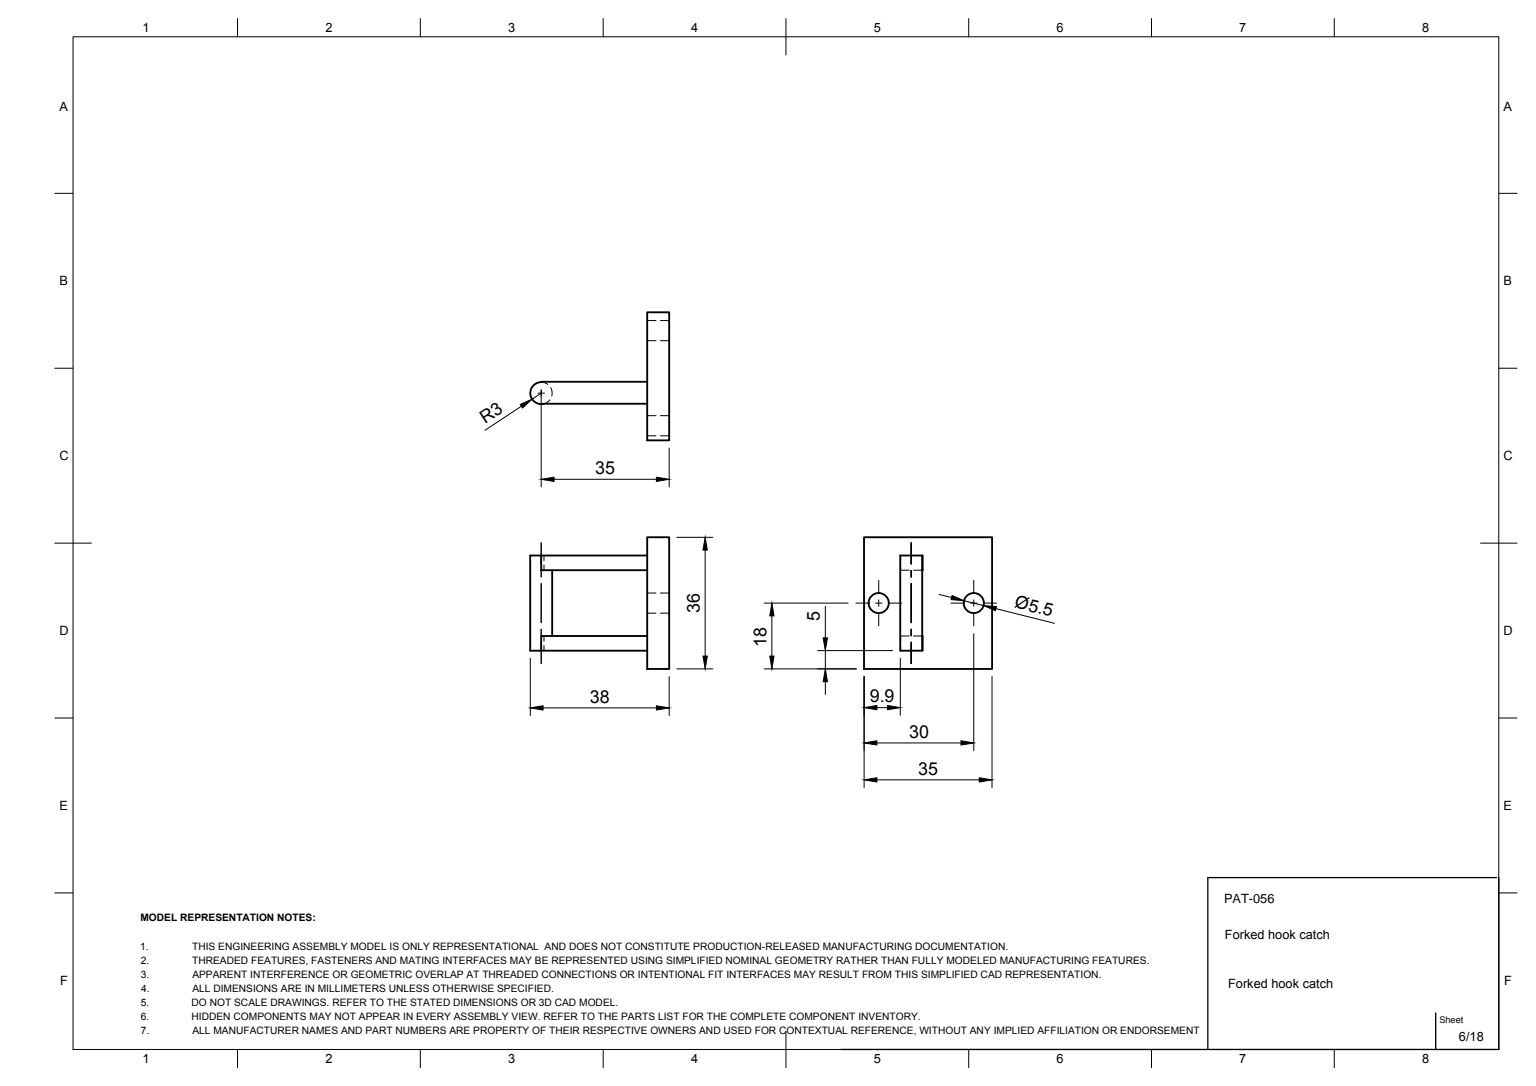
ISO-10303-21;
HEADER;
/* Generated by software containing ST-Developer
 * from STEP Tools, Inc. (www.steptools.com) 
 */

FILE_DESCRIPTION(
/* description */ ('Hook toggle clamp'),
/* implementation_level */ '2;1');

FILE_NAME(
/* name */ 'Forked hook catch.step',
/* time_stamp */ '2026-10-27T21:56:56-07:00',
/* author */ (''),
/* organization */ (''),
/* preprocessor_version */ 'ST-DEVELOPER v20.2',
/* originating_system */ 'Autodesk Translation Framework v15.17.0.0',
/* authorisation */ '');

FILE_SCHEMA (('AUTOMOTIVE_DESIGN { 1 0 10303 214 3 1 1 }'));
ENDSEC;

DATA;
#10=MECHANICAL_DESIGN_GEOMETRIC_PRESENTATION_REPRESENTATION('',(#191),#5458);
#157=SHAPE_REPRESENTATION_RELATIONSHIP('SRR','None',#5538,#174);
#174=ADVANCED_BREP_SHAPE_REPRESENTATION('',(#208),#5440);
#191=STYLED_ITEM('',(#5731),#208);
#208=MANIFOLD_SOLID_BREP('Body1',#2972);
#237=FACE_BOUND('',#641,.T.);
#238=FACE_BOUND('',#642,.T.);
#239=FACE_BOUND('',#643,.T.);
#240=FACE_BOUND('',#644,.T.);
#241=FACE_BOUND('',#646,.T.);
#242=FACE_BOUND('',#647,.T.);
#312=PLANE('',#3244);
#313=PLANE('',#3252);
#314=PLANE('',#3253);
#315=PLANE('',#3254);
#316=PLANE('',#3255);
#317=PLANE('',#3256);
#318=PLANE('',#3257);
#319=PLANE('',#3258);
#320=PLANE('',#3259);
#321=PLANE('',#3260);
#322=PLANE('',#3261);
#323=PLANE('',#3262);
#324=PLANE('',#3263);
#325=PLANE('',#3264);
#326=PLANE('',#3265);
#327=PLANE('',#3266);
#435=FACE_OUTER_BOUND('',#623,.T.);
#436=FACE_OUTER_BOUND('',#624,.T.);
#437=FACE_OUTER_BOUND('',#625,.T.);
#438=FACE_OUTER_BOUND('',#626,.T.);
#439=FACE_OUTER_BOUND('',#627,.T.);
#440=FACE_OUTER_BOUND('',#628,.T.);
#441=FACE_OUTER_BOUND('',#629,.T.);
#442=FACE_OUTER_BOUND('',#630,.T.);
#443=FACE_OUTER_BOUND('',#631,.T.);
#444=FACE_OUTER_BOUND('',#632,.T.);
#445=FACE_OUTER_BOUND('',#633,.T.);
#446=FACE_OUTER_BOUND('',#634,.T.);
#447=FACE_OUTER_BOUND('',#635,.T.);
#448=FACE_OUTER_BOUND('',#636,.T.);
#449=FACE_OUTER_BOUND('',#637,.T.);
#450=FACE_OUTER_BOUND('',#638,.T.);
#451=FACE_OUTER_BOUND('',#639,.T.);
#452=FACE_OUTER_BOUND('',#640,.T.);
#453=FACE_OUTER_BOUND('',#645,.T.);
#623=EDGE_LOOP('',(#2197,#2198,#2199,#2200));
#624=EDGE_LOOP('',(#2201,#2202,#2203,#2204));
#625=EDGE_LOOP('',(#2205,#2206,#2207,#2208,#2209));
#626=EDGE_LOOP('',(#2210,#2211,#2212,#2213,#2214,#2215,#2216,#2217,#2218,
#2219,#2220,#2221));
#627=EDGE_LOOP('',(#2222,#2223,#2224,#2225,#2226,#2227));
#628=EDGE_LOOP('',(#2228,#2229,#2230,#2231));
#629=EDGE_LOOP('',(#2232,#2233,#2234,#2235));
#630=EDGE_LOOP('',(#2236,#2237,#2238,#2239));
#631=EDGE_LOOP('',(#2240,#2241,#2242,#2243,#2244));
#632=EDGE_LOOP('',(#2245,#2246,#2247,#2248));
#633=EDGE_LOOP('',(#2249,#2250,#2251,#2252,#2253,#2254));
#634=EDGE_LOOP('',(#2255,#2256,#2257,#2258));
#635=EDGE_LOOP('',(#2259,#2260,#2261,#2262));
#636=EDGE_LOOP('',(#2263,#2264,#2265,#2266));
#637=EDGE_LOOP('',(#2267,#2268,#2269,#2270));
#638=EDGE_LOOP('',(#2271,#2272,#2273,#2274));
#639=EDGE_LOOP('',(#2275,#2276,#2277,#2278));
#640=EDGE_LOOP('',(#2279,#2280,#2281,#2282));
#641=EDGE_LOOP('',(#2283));
#642=EDGE_LOOP('',(#2284));
#643=EDGE_LOOP('',(#2285,#2286,#2287,#2288));
#644=EDGE_LOOP('',(#2289,#2290,#2291,#2292));
#645=EDGE_LOOP('',(#2293,#2294,#2295,#2296));
#646=EDGE_LOOP('',(#2297));
#647=EDGE_LOOP('',(#2298));
#872=LINE('',#4644,#1109);
#873=LINE('',#4650,#1110);
#874=LINE('',#4657,#1111);
#875=LINE('',#4659,#1112);
#876=LINE('',#4661,#1113);
#877=LINE('',#4662,#1114);
#878=LINE('',#4665,#1115);
#879=LINE('',#4667,#1116);
#880=LINE('',#4671,#1117);
#881=LINE('',#4675,#1118);
#882=LINE('',#4679,#1119);
#883=LINE('',#4684,#1120);
#884=LINE('',#4686,#1121);
#885=LINE('',#4688,#1122);
#886=LINE('',#4689,#1123);
#887=LINE('',#4691,#1124);
#888=LINE('',#4693,#1125);
#889=LINE('',#4695,#1126);
#890=LINE('',#4698,#1127);
#891=LINE('',#4700,#1128);
#892=LINE('',#4702,#1129);
#893=LINE('',#4703,#1130);
#894=LINE('',#4706,#1131);
#895=LINE('',#4707,#1132);
#896=LINE('',#4710,#1133);
#897=LINE('',#4712,#1134);
#898=LINE('',#4713,#1135);
#899=LINE('',#4715,#1136);
#900=LINE('',#4717,#1137);
#901=LINE('',#4721,#1138);
#902=LINE('',#4723,#1139);
#903=LINE('',#4725,#1140);
#904=LINE('',#4726,#1141);
#905=LINE('',#4729,#1142);
#906=LINE('',#4731,#1143);
#907=LINE('',#4732,#1144);
#908=LINE('',#4735,#1145);
#909=LINE('',#4737,#1146);
#910=LINE('',#4738,#1147);
#911=LINE('',#4740,#1148);
#912=LINE('',#4741,#1149);
#1109=VECTOR('',#3716,0.275);
#1110=VECTOR('',#3723,0.274999999999999);
#1111=VECTOR('',#3730,1.);
#1112=VECTOR('',#3731,1.);
#1113=VECTOR('',#3732,1.);
#1114=VECTOR('',#3733,1.);
#1115=VECTOR('',#3736,1.);
#1116=VECTOR('',#3737,1.);
#1117=VECTOR('',#3740,0.300000000000001);
#1118=VECTOR('',#3743,1.);
#1119=VECTOR('',#3746,1.);
#1120=VECTOR('',#3753,1.);
#1121=VECTOR('',#3754,1.);
#1122=VECTOR('',#3755,1.);
#1123=VECTOR('',#3756,1.);
#1124=VECTOR('',#3759,1.);
#1125=VECTOR('',#3762,1.);
#1126=VECTOR('',#3765,1.);
#1127=VECTOR('',#3768,1.);
#1128=VECTOR('',#3769,1.);
#1129=VECTOR('',#3770,1.);
#1130=VECTOR('',#3771,1.);
#1131=VECTOR('',#3774,1.);
#1132=VECTOR('',#3775,1.);
#1133=VECTOR('',#3778,1.);
#1134=VECTOR('',#3779,1.);
#1135=VECTOR('',#3780,1.);
#1136=VECTOR('',#3783,1.);
#1137=VECTOR('',#3786,1.);
#1138=VECTOR('',#3789,1.);
#1139=VECTOR('',#3790,1.);
#1140=VECTOR('',#3791,1.);
#1141=VECTOR('',#3792,1.);
#1142=VECTOR('',#3795,1.);
#1143=VECTOR('',#3796,1.);
#1144=VECTOR('',#3797,1.);
#1145=VECTOR('',#3800,1.);
#1146=VECTOR('',#3801,1.);
#1147=VECTOR('',#3802,1.);
#1148=VECTOR('',#3805,1.);
#1149=VECTOR('',#3806,1.);
#1284=CIRCLE('',#3239,0.275);
#1285=CIRCLE('',#3240,0.275);
#1286=CIRCLE('',#3242,0.274999999999999);
#1287=CIRCLE('',#3243,0.274999999999999);
#1288=CIRCLE('',#3245,0.300000000000001);
#1289=CIRCLE('',#3247,0.300000000000001);
#1290=CIRCLE('',#3248,0.300000000000001);
#1291=CIRCLE('',#3249,0.300000000000001);
#1292=CIRCLE('',#3250,0.300000000000001);
#1293=CIRCLE('',#3251,0.300000000000001);
#1447=VERTEX_POINT('',#4641);
#1448=VERTEX_POINT('',#4643);
#1449=VERTEX_POINT('',#4647);
#1450=VERTEX_POINT('',#4649);
#1451=VERTEX_POINT('',#4653);
#1452=VERTEX_POINT('',#4654);
#1453=VERTEX_POINT('',#4656);
#1454=VERTEX_POINT('',#4658);
#1455=VERTEX_POINT('',#4660);
#1456=VERTEX_POINT('',#4664);
#1457=VERTEX_POINT('',#4666);
#1458=VERTEX_POINT('',#4668);
#1459=VERTEX_POINT('',#4670);
#1460=VERTEX_POINT('',#4672);
#1461=VERTEX_POINT('',#4674);
#1462=VERTEX_POINT('',#4676);
#1463=VERTEX_POINT('',#4678);
#1464=VERTEX_POINT('',#4683);
#1465=VERTEX_POINT('',#4685);
#1466=VERTEX_POINT('',#4687);
#1467=VERTEX_POINT('',#4697);
#1468=VERTEX_POINT('',#4699);
#1469=VERTEX_POINT('',#4701);
#1470=VERTEX_POINT('',#4705);
#1471=VERTEX_POINT('',#4709);
#1472=VERTEX_POINT('',#4711);
#1473=VERTEX_POINT('',#4719);
#1474=VERTEX_POINT('',#4720);
#1475=VERTEX_POINT('',#4722);
#1476=VERTEX_POINT('',#4724);
#1477=VERTEX_POINT('',#4728);
#1478=VERTEX_POINT('',#4730);
#1479=VERTEX_POINT('',#4734);
#1480=VERTEX_POINT('',#4736);
#1725=EDGE_CURVE('',#1447,#1447,#1284,.T.);
#1726=EDGE_CURVE('',#1447,#1448,#872,.T.);
#1727=EDGE_CURVE('',#1448,#1448,#1285,.T.);
#1728=EDGE_CURVE('',#1449,#1449,#1286,.T.);
#1729=EDGE_CURVE('',#1449,#1450,#873,.T.);
#1730=EDGE_CURVE('',#1450,#1450,#1287,.T.);
#1731=EDGE_CURVE('',#1451,#1452,#1288,.T.);
#1732=EDGE_CURVE('',#1452,#1453,#874,.T.);
#1733=EDGE_CURVE('',#1454,#1453,#875,.T.);
#1734=EDGE_CURVE('',#1454,#1455,#876,.T.);
#1735=EDGE_CURVE('',#1455,#1451,#877,.T.);
#1736=EDGE_CURVE('',#1452,#1456,#878,.T.);
#1737=EDGE_CURVE('',#1457,#1451,#879,.T.);
#1738=EDGE_CURVE('',#1458,#1457,#1289,.T.);
#1739=EDGE_CURVE('',#1458,#1459,#880,.T.);
#1740=EDGE_CURVE('',#1459,#1460,#1290,.T.);
#1741=EDGE_CURVE('',#1461,#1460,#881,.T.);
#1742=EDGE_CURVE('',#1462,#1461,#1291,.T.);
#1743=EDGE_CURVE('',#1463,#1462,#882,.T.);
#1744=EDGE_CURVE('',#1463,#1459,#1292,.T.);
#1745=EDGE_CURVE('',#1456,#1458,#1293,.T.);
#1746=EDGE_CURVE('',#1457,#1464,#883,.T.);
#1747=EDGE_CURVE('',#1464,#1465,#884,.T.);
#1748=EDGE_CURVE('',#1466,#1465,#885,.T.);
#1749=EDGE_CURVE('',#1466,#1456,#886,.T.);
#1750=EDGE_CURVE('',#1455,#1464,#887,.T.);
#1751=EDGE_CURVE('',#1465,#1454,#888,.T.);
#1752=EDGE_CURVE('',#1453,#1466,#889,.T.);
#1753=EDGE_CURVE('',#1461,#1467,#890,.T.);
#1754=EDGE_CURVE('',#1467,#1468,#891,.T.);
#1755=EDGE_CURVE('',#1469,#1468,#892,.T.);
#1756=EDGE_CURVE('',#1469,#1462,#893,.T.);
#1757=EDGE_CURVE('',#1470,#1460,#894,.T.);
#1758=EDGE_CURVE('',#1470,#1467,#895,.T.);
#1759=EDGE_CURVE('',#1463,#1471,#896,.T.);
#1760=EDGE_CURVE('',#1472,#1471,#897,.T.);
#1761=EDGE_CURVE('',#1472,#1470,#898,.T.);
#1762=EDGE_CURVE('',#1468,#1472,#899,.T.);
#1763=EDGE_CURVE('',#1471,#1469,#900,.T.);
#1764=EDGE_CURVE('',#1473,#1474,#901,.T.);
#1765=EDGE_CURVE('',#1474,#1475,#902,.T.);
#1766=EDGE_CURVE('',#1476,#1475,#903,.T.);
#1767=EDGE_CURVE('',#1473,#1476,#904,.T.);
#1768=EDGE_CURVE('',#1477,#1473,#905,.T.);
#1769=EDGE_CURVE('',#1478,#1476,#906,.T.);
#1770=EDGE_CURVE('',#1477,#1478,#907,.T.);
#1771=EDGE_CURVE('',#1479,#1477,#908,.T.);
#1772=EDGE_CURVE('',#1480,#1478,#909,.T.);
#1773=EDGE_CURVE('',#1479,#1480,#910,.T.);
#1774=EDGE_CURVE('',#1474,#1479,#911,.T.);
#1775=EDGE_CURVE('',#1475,#1480,#912,.T.);
#2197=ORIENTED_EDGE('',*,*,#1725,.F.);
#2198=ORIENTED_EDGE('',*,*,#1726,.T.);
#2199=ORIENTED_EDGE('',*,*,#1727,.F.);
#2200=ORIENTED_EDGE('',*,*,#1726,.F.);
#2201=ORIENTED_EDGE('',*,*,#1728,.F.);
#2202=ORIENTED_EDGE('',*,*,#1729,.T.);
#2203=ORIENTED_EDGE('',*,*,#1730,.F.);
#2204=ORIENTED_EDGE('',*,*,#1729,.F.);
#2205=ORIENTED_EDGE('',*,*,#1731,.T.);
#2206=ORIENTED_EDGE('',*,*,#1732,.T.);
#2207=ORIENTED_EDGE('',*,*,#1733,.F.);
#2208=ORIENTED_EDGE('',*,*,#1734,.T.);
#2209=ORIENTED_EDGE('',*,*,#1735,.T.);
#2210=ORIENTED_EDGE('',*,*,#1736,.F.);
#2211=ORIENTED_EDGE('',*,*,#1731,.F.);
#2212=ORIENTED_EDGE('',*,*,#1737,.F.);
#2213=ORIENTED_EDGE('',*,*,#1738,.F.);
#2214=ORIENTED_EDGE('',*,*,#1739,.T.);
#2215=ORIENTED_EDGE('',*,*,#1740,.T.);
#2216=ORIENTED_EDGE('',*,*,#1741,.F.);
#2217=ORIENTED_EDGE('',*,*,#1742,.F.);
#2218=ORIENTED_EDGE('',*,*,#1743,.F.);
#2219=ORIENTED_EDGE('',*,*,#1744,.T.);
#2220=ORIENTED_EDGE('',*,*,#1739,.F.);
#2221=ORIENTED_EDGE('',*,*,#1745,.F.);
#2222=ORIENTED_EDGE('',*,*,#1746,.T.);
#2223=ORIENTED_EDGE('',*,*,#1747,.T.);
#2224=ORIENTED_EDGE('',*,*,#1748,.F.);
#2225=ORIENTED_EDGE('',*,*,#1749,.T.);
#2226=ORIENTED_EDGE('',*,*,#1745,.T.);
#2227=ORIENTED_EDGE('',*,*,#1738,.T.);
#2228=ORIENTED_EDGE('',*,*,#1737,.T.);
#2229=ORIENTED_EDGE('',*,*,#1735,.F.);
#2230=ORIENTED_EDGE('',*,*,#1750,.T.);
#2231=ORIENTED_EDGE('',*,*,#1746,.F.);
#2232=ORIENTED_EDGE('',*,*,#1751,.F.);
#2233=ORIENTED_EDGE('',*,*,#1747,.F.);
#2234=ORIENTED_EDGE('',*,*,#1750,.F.);
#2235=ORIENTED_EDGE('',*,*,#1734,.F.);
#2236=ORIENTED_EDGE('',*,*,#1736,.T.);
#2237=ORIENTED_EDGE('',*,*,#1749,.F.);
#2238=ORIENTED_EDGE('',*,*,#1752,.F.);
#2239=ORIENTED_EDGE('',*,*,#1732,.F.);
#2240=ORIENTED_EDGE('',*,*,#1742,.T.);
#2241=ORIENTED_EDGE('',*,*,#1753,.T.);
#2242=ORIENTED_EDGE('',*,*,#1754,.T.);
#2243=ORIENTED_EDGE('',*,*,#1755,.F.);
#2244=ORIENTED_EDGE('',*,*,#1756,.T.);
#2245=ORIENTED_EDGE('',*,*,#1741,.T.);
#2246=ORIENTED_EDGE('',*,*,#1757,.F.);
#2247=ORIENTED_EDGE('',*,*,#1758,.T.);
#2248=ORIENTED_EDGE('',*,*,#1753,.F.);
#2249=ORIENTED_EDGE('',*,*,#1759,.T.);
#2250=ORIENTED_EDGE('',*,*,#1760,.F.);
#2251=ORIENTED_EDGE('',*,*,#1761,.T.);
#2252=ORIENTED_EDGE('',*,*,#1757,.T.);
#2253=ORIENTED_EDGE('',*,*,#1740,.F.);
#2254=ORIENTED_EDGE('',*,*,#1744,.F.);
#2255=ORIENTED_EDGE('',*,*,#1762,.F.);
#2256=ORIENTED_EDGE('',*,*,#1754,.F.);
#2257=ORIENTED_EDGE('',*,*,#1758,.F.);
#2258=ORIENTED_EDGE('',*,*,#1761,.F.);
#2259=ORIENTED_EDGE('',*,*,#1743,.T.);
#2260=ORIENTED_EDGE('',*,*,#1756,.F.);
#2261=ORIENTED_EDGE('',*,*,#1763,.F.);
#2262=ORIENTED_EDGE('',*,*,#1759,.F.);
#2263=ORIENTED_EDGE('',*,*,#1764,.T.);
#2264=ORIENTED_EDGE('',*,*,#1765,.T.);
#2265=ORIENTED_EDGE('',*,*,#1766,.F.);
#2266=ORIENTED_EDGE('',*,*,#1767,.F.);
#2267=ORIENTED_EDGE('',*,*,#1768,.T.);
#2268=ORIENTED_EDGE('',*,*,#1767,.T.);
#2269=ORIENTED_EDGE('',*,*,#1769,.F.);
#2270=ORIENTED_EDGE('',*,*,#1770,.F.);
#2271=ORIENTED_EDGE('',*,*,#1771,.T.);
#2272=ORIENTED_EDGE('',*,*,#1770,.T.);
#2273=ORIENTED_EDGE('',*,*,#1772,.F.);
#2274=ORIENTED_EDGE('',*,*,#1773,.F.);
#2275=ORIENTED_EDGE('',*,*,#1774,.T.);
#2276=ORIENTED_EDGE('',*,*,#1773,.T.);
#2277=ORIENTED_EDGE('',*,*,#1775,.F.);
#2278=ORIENTED_EDGE('',*,*,#1765,.F.);
#2279=ORIENTED_EDGE('',*,*,#1775,.T.);
#2280=ORIENTED_EDGE('',*,*,#1772,.T.);
#2281=ORIENTED_EDGE('',*,*,#1769,.T.);
#2282=ORIENTED_EDGE('',*,*,#1766,.T.);
#2283=ORIENTED_EDGE('',*,*,#1727,.T.);
#2284=ORIENTED_EDGE('',*,*,#1730,.T.);
#2285=ORIENTED_EDGE('',*,*,#1751,.T.);
#2286=ORIENTED_EDGE('',*,*,#1733,.T.);
#2287=ORIENTED_EDGE('',*,*,#1752,.T.);
#2288=ORIENTED_EDGE('',*,*,#1748,.T.);
#2289=ORIENTED_EDGE('',*,*,#1762,.T.);
#2290=ORIENTED_EDGE('',*,*,#1760,.T.);
#2291=ORIENTED_EDGE('',*,*,#1763,.T.);
#2292=ORIENTED_EDGE('',*,*,#1755,.T.);
#2293=ORIENTED_EDGE('',*,*,#1774,.F.);
#2294=ORIENTED_EDGE('',*,*,#1764,.F.);
#2295=ORIENTED_EDGE('',*,*,#1768,.F.);
#2296=ORIENTED_EDGE('',*,*,#1771,.F.);
#2297=ORIENTED_EDGE('',*,*,#1725,.T.);
#2298=ORIENTED_EDGE('',*,*,#1728,.T.);
#2756=CYLINDRICAL_SURFACE('',#3238,0.275);
#2757=CYLINDRICAL_SURFACE('',#3241,0.274999999999999);
#2758=CYLINDRICAL_SURFACE('',#3246,0.300000000000001);
#2839=ADVANCED_FACE('',(#435),#2756,.F.);
#2840=ADVANCED_FACE('',(#436),#2757,.F.);
#2841=ADVANCED_FACE('',(#437),#312,.F.);
#2842=ADVANCED_FACE('',(#438),#2758,.T.);
#2843=ADVANCED_FACE('',(#439),#313,.T.);
#2844=ADVANCED_FACE('',(#440),#314,.T.);
#2845=ADVANCED_FACE('',(#441),#315,.T.);
#2846=ADVANCED_FACE('',(#442),#316,.T.);
#2847=ADVANCED_FACE('',(#443),#317,.T.);
#2848=ADVANCED_FACE('',(#444),#318,.T.);
#2849=ADVANCED_FACE('',(#445),#319,.F.);
#2850=ADVANCED_FACE('',(#446),#320,.T.);
#2851=ADVANCED_FACE('',(#447),#321,.T.);
#2852=ADVANCED_FACE('',(#448),#322,.T.);
#2853=ADVANCED_FACE('',(#449),#323,.T.);
#2854=ADVANCED_FACE('',(#450),#324,.T.);
#2855=ADVANCED_FACE('',(#451),#325,.T.);
#2856=ADVANCED_FACE('',(#452,#237,#238,#239,#240),#326,.T.);
#2857=ADVANCED_FACE('',(#453,#241,#242),#327,.F.);
#2972=CLOSED_SHELL('',(#2839,#2840,#2841,#2842,#2843,#2844,#2845,#2846,
#2847,#2848,#2849,#2850,#2851,#2852,#2853,#2854,#2855,#2856,#2857));
#3237=AXIS2_PLACEMENT_3D('',#4639,#3710,#3711);
#3238=AXIS2_PLACEMENT_3D('',#4640,#3712,#3713);
#3239=AXIS2_PLACEMENT_3D('',#4642,#3714,#3715);
#3240=AXIS2_PLACEMENT_3D('',#4645,#3717,#3718);
#3241=AXIS2_PLACEMENT_3D('',#4646,#3719,#3720);
#3242=AXIS2_PLACEMENT_3D('',#4648,#3721,#3722);
#3243=AXIS2_PLACEMENT_3D('',#4651,#3724,#3725);
#3244=AXIS2_PLACEMENT_3D('',#4652,#3726,#3727);
#3245=AXIS2_PLACEMENT_3D('',#4655,#3728,#3729);
#3246=AXIS2_PLACEMENT_3D('',#4663,#3734,#3735);
#3247=AXIS2_PLACEMENT_3D('',#4669,#3738,#3739);
#3248=AXIS2_PLACEMENT_3D('',#4673,#3741,#3742);
#3249=AXIS2_PLACEMENT_3D('',#4677,#3744,#3745);
#3250=AXIS2_PLACEMENT_3D('',#4680,#3747,#3748);
#3251=AXIS2_PLACEMENT_3D('',#4681,#3749,#3750);
#3252=AXIS2_PLACEMENT_3D('',#4682,#3751,#3752);
#3253=AXIS2_PLACEMENT_3D('',#4690,#3757,#3758);
#3254=AXIS2_PLACEMENT_3D('',#4692,#3760,#3761);
#3255=AXIS2_PLACEMENT_3D('',#4694,#3763,#3764);
#3256=AXIS2_PLACEMENT_3D('',#4696,#3766,#3767);
#3257=AXIS2_PLACEMENT_3D('',#4704,#3772,#3773);
#3258=AXIS2_PLACEMENT_3D('',#4708,#3776,#3777);
#3259=AXIS2_PLACEMENT_3D('',#4714,#3781,#3782);
#3260=AXIS2_PLACEMENT_3D('',#4716,#3784,#3785);
#3261=AXIS2_PLACEMENT_3D('',#4718,#3787,#3788);
#3262=AXIS2_PLACEMENT_3D('',#4727,#3793,#3794);
#3263=AXIS2_PLACEMENT_3D('',#4733,#3798,#3799);
#3264=AXIS2_PLACEMENT_3D('',#4739,#3803,#3804);
#3265=AXIS2_PLACEMENT_3D('',#4742,#3807,#3808);
#3266=AXIS2_PLACEMENT_3D('',#4743,#3809,#3810);
#3710=DIRECTION('axis',(0.,0.,1.));
#3711=DIRECTION('refdir',(1.,0.,0.));
#3712=DIRECTION('center_axis',(0.,0.,1.));
#3713=DIRECTION('ref_axis',(1.,0.,0.));
#3714=DIRECTION('center_axis',(0.,0.,1.));
#3715=DIRECTION('ref_axis',(1.,0.,0.));
#3716=DIRECTION('',(0.,0.,1.));
#3717=DIRECTION('center_axis',(0.,0.,-1.));
#3718=DIRECTION('ref_axis',(1.,0.,0.));
#3719=DIRECTION('center_axis',(0.,0.,1.));
#3720=DIRECTION('ref_axis',(1.,0.,0.));
#3721=DIRECTION('center_axis',(0.,0.,1.));
#3722=DIRECTION('ref_axis',(1.,0.,0.));
#3723=DIRECTION('',(0.,0.,1.));
#3724=DIRECTION('center_axis',(0.,0.,-1.));
#3725=DIRECTION('ref_axis',(1.,0.,0.));
#3726=DIRECTION('center_axis',(0.,1.,0.));
#3727=DIRECTION('ref_axis',(1.,0.,0.));
#3728=DIRECTION('center_axis',(0.,1.,0.));
#3729=DIRECTION('ref_axis',(1.,0.,0.));
#3730=DIRECTION('',(0.,0.,-1.));
#3731=DIRECTION('',(-1.,0.,0.));
#3732=DIRECTION('',(0.,0.,1.));
#3733=DIRECTION('',(-1.,0.,0.));
#3734=DIRECTION('center_axis',(0.,1.,0.));
#3735=DIRECTION('ref_axis',(1.,0.,0.));
#3736=DIRECTION('',(0.,1.,0.));
#3737=DIRECTION('',(0.,-1.,0.));
#3738=DIRECTION('center_axis',(0.,1.,0.));
#3739=DIRECTION('ref_axis',(1.,0.,0.));
#3740=DIRECTION('',(0.,-1.,0.));
#3741=DIRECTION('center_axis',(0.,1.,0.));
#3742=DIRECTION('ref_axis',(1.,0.,0.));
#3743=DIRECTION('',(0.,-1.,0.));
#3744=DIRECTION('center_axis',(0.,-1.,0.));
#3745=DIRECTION('ref_axis',(1.,0.,0.));
#3746=DIRECTION('',(0.,1.,0.));
#3747=DIRECTION('center_axis',(0.,1.,0.));
#3748=DIRECTION('ref_axis',(1.,0.,0.));
#3749=DIRECTION('center_axis',(0.,1.,0.));
#3750=DIRECTION('ref_axis',(1.,0.,0.));
#3751=DIRECTION('center_axis',(0.,1.,0.));
#3752=DIRECTION('ref_axis',(0.,0.,1.));
#3753=DIRECTION('',(1.,0.,0.));
#3754=DIRECTION('',(0.,0.,-1.));
#3755=DIRECTION('',(1.,0.,0.));
#3756=DIRECTION('',(0.,0.,1.));
#3757=DIRECTION('center_axis',(0.,0.,1.));
#3758=DIRECTION('ref_axis',(1.,0.,0.));
#3759=DIRECTION('',(0.,1.,0.));
#3760=DIRECTION('center_axis',(1.,0.,0.));
#3761=DIRECTION('ref_axis',(0.,0.,-1.));
#3762=DIRECTION('',(0.,-1.,0.));
#3763=DIRECTION('center_axis',(-1.,0.,0.));
#3764=DIRECTION('ref_axis',(0.,0.,1.));
#3765=DIRECTION('',(0.,1.,0.));
#3766=DIRECTION('center_axis',(0.,1.,0.));
#3767=DIRECTION('ref_axis',(0.,0.,1.));
#3768=DIRECTION('',(1.,0.,0.));
#3769=DIRECTION('',(0.,0.,-1.));
#3770=DIRECTION('',(1.,0.,0.));
#3771=DIRECTION('',(0.,0.,1.));
#3772=DIRECTION('center_axis',(0.,0.,1.));
#3773=DIRECTION('ref_axis',(1.,0.,0.));
#3774=DIRECTION('',(-1.,0.,0.));
#3775=DIRECTION('',(0.,1.,0.));
#3776=DIRECTION('center_axis',(0.,1.,0.));
#3777=DIRECTION('ref_axis',(1.,0.,0.));
#3778=DIRECTION('',(0.,0.,-1.));
#3779=DIRECTION('',(-1.,0.,0.));
#3780=DIRECTION('',(0.,0.,1.));
#3781=DIRECTION('center_axis',(1.,0.,0.));
#3782=DIRECTION('ref_axis',(0.,0.,-1.));
#3783=DIRECTION('',(0.,-1.,0.));
#3784=DIRECTION('center_axis',(-1.,0.,0.));
#3785=DIRECTION('ref_axis',(0.,0.,1.));
#3786=DIRECTION('',(0.,1.,0.));
#3787=DIRECTION('center_axis',(0.,1.,0.));
#3788=DIRECTION('ref_axis',(-1.,0.,0.));
#3789=DIRECTION('',(-1.,0.,0.));
#3790=DIRECTION('',(0.,0.,1.));
#3791=DIRECTION('',(-1.,0.,0.));
#3792=DIRECTION('',(0.,0.,1.));
#3793=DIRECTION('center_axis',(1.,0.,0.));
#3794=DIRECTION('ref_axis',(0.,1.,0.));
#3795=DIRECTION('',(0.,1.,0.));
#3796=DIRECTION('',(0.,1.,0.));
#3797=DIRECTION('',(0.,0.,1.));
#3798=DIRECTION('center_axis',(0.,-1.,0.));
#3799=DIRECTION('ref_axis',(1.,0.,0.));
#3800=DIRECTION('',(1.,0.,0.));
#3801=DIRECTION('',(1.,0.,0.));
#3802=DIRECTION('',(0.,0.,1.));
#3803=DIRECTION('center_axis',(-1.,0.,0.));
#3804=DIRECTION('ref_axis',(0.,-1.,0.));
#3805=DIRECTION('',(0.,-1.,0.));
#3806=DIRECTION('',(0.,-1.,0.));
#3807=DIRECTION('center_axis',(0.,0.,1.));
#3808=DIRECTION('ref_axis',(1.,0.,0.));
#3809=DIRECTION('center_axis',(0.,0.,1.));
#3810=DIRECTION('ref_axis',(1.,0.,0.));
#4639=CARTESIAN_POINT('',(0.,0.,0.));
#4640=CARTESIAN_POINT('Origin',(14.4,0.,-0.1));
#4641=CARTESIAN_POINT('',(14.125,-3.36777869765523E-17,0.));
#4642=CARTESIAN_POINT('Origin',(14.4,0.,0.));
#4643=CARTESIAN_POINT('',(14.125,3.36777869765523E-17,0.6));
#4644=CARTESIAN_POINT('',(14.125,-3.36777869765523E-17,-0.1));
#4645=CARTESIAN_POINT('Origin',(14.4,0.,0.6));
#4646=CARTESIAN_POINT('Origin',(17.,0.,-0.1));
#4647=CARTESIAN_POINT('',(16.725,-3.3677786976552E-17,0.));
#4648=CARTESIAN_POINT('Origin',(17.,0.,0.));
#4649=CARTESIAN_POINT('',(16.725,3.3677786976552E-17,0.6));
#4650=CARTESIAN_POINT('',(16.725,-3.3677786976552E-17,-0.1));
#4651=CARTESIAN_POINT('Origin',(17.,0.,0.6));
#4652=CARTESIAN_POINT('Origin',(15.3,0.9,2.));
#4653=CARTESIAN_POINT('',(15.59,0.9,3.5));
#4654=CARTESIAN_POINT('',(15.,0.9,3.42318854252131));
#4655=CARTESIAN_POINT('Origin',(15.29,0.9,3.5));
#4656=CARTESIAN_POINT('',(15.,0.9,0.6));
#4657=CARTESIAN_POINT('',(15.,0.9,3.5));
#4658=CARTESIAN_POINT('',(15.6,0.9,0.6));
#4659=CARTESIAN_POINT('',(15.525,0.9,0.6));
#4660=CARTESIAN_POINT('',(15.6,0.9,3.5));
#4661=CARTESIAN_POINT('',(15.6,0.9,0.5));
#4662=CARTESIAN_POINT('',(15.6,0.9,3.5));
#4663=CARTESIAN_POINT('Origin',(15.29,0.9,3.5));
#4664=CARTESIAN_POINT('',(15.,1.3,3.42318854252131));
#4665=CARTESIAN_POINT('',(15.,0.9,3.42318854252131));
#4666=CARTESIAN_POINT('',(15.59,1.3,3.5));
#4667=CARTESIAN_POINT('',(15.59,0.9,3.5));
#4668=CARTESIAN_POINT('',(14.99,1.3,3.5));
#4669=CARTESIAN_POINT('Origin',(15.29,1.3,3.5));
#4670=CARTESIAN_POINT('',(14.99,-1.3,3.5));
#4671=CARTESIAN_POINT('',(14.99,0.9,3.5));
#4672=CARTESIAN_POINT('',(15.59,-1.3,3.5));
#4673=CARTESIAN_POINT('Origin',(15.29,-1.3,3.5));
#4674=CARTESIAN_POINT('',(15.59,-0.9,3.5));
#4675=CARTESIAN_POINT('',(15.59,-1.3,3.5));
#4676=CARTESIAN_POINT('',(15.,-0.9,3.42318854252131));
#4677=CARTESIAN_POINT('Origin',(15.29,-0.9,3.5));
#4678=CARTESIAN_POINT('',(15.,-1.3,3.42318854252131));
#4679=CARTESIAN_POINT('',(15.,-1.3,3.42318854252131));
#4680=CARTESIAN_POINT('Origin',(15.29,-1.3,3.5));
#4681=CARTESIAN_POINT('Origin',(15.29,1.3,3.5));
#4682=CARTESIAN_POINT('Origin',(15.3,1.3,2.));
#4683=CARTESIAN_POINT('',(15.6,1.3,3.5));
#4684=CARTESIAN_POINT('',(15.6,1.3,3.5));
#4685=CARTESIAN_POINT('',(15.6,1.3,0.6));
#4686=CARTESIAN_POINT('',(15.6,1.3,0.5));
#4687=CARTESIAN_POINT('',(15.,1.3,0.6));
#4688=CARTESIAN_POINT('',(15.525,1.3,0.6));
#4689=CARTESIAN_POINT('',(15.,1.3,3.5));
#4690=CARTESIAN_POINT('Origin',(15.,0.9,3.5));
#4691=CARTESIAN_POINT('',(15.6,0.9,3.5));
#4692=CARTESIAN_POINT('Origin',(15.6,0.9,3.5));
#4693=CARTESIAN_POINT('',(15.6,0.45,0.6));
#4694=CARTESIAN_POINT('Origin',(15.,0.9,0.5));
#4695=CARTESIAN_POINT('',(15.,0.45,0.6));
#4696=CARTESIAN_POINT('Origin',(15.3,-0.9,2.));
#4697=CARTESIAN_POINT('',(15.6,-0.9,3.5));
#4698=CARTESIAN_POINT('',(15.6,-0.9,3.5));
#4699=CARTESIAN_POINT('',(15.6,-0.9,0.6));
#4700=CARTESIAN_POINT('',(15.6,-0.9,0.5));
#4701=CARTESIAN_POINT('',(15.,-0.9,0.6));
#4702=CARTESIAN_POINT('',(15.525,-0.9,0.6));
#4703=CARTESIAN_POINT('',(15.,-0.9,3.5));
#4704=CARTESIAN_POINT('Origin',(15.,-1.3,3.5));
#4705=CARTESIAN_POINT('',(15.6,-1.3,3.5));
#4706=CARTESIAN_POINT('',(15.6,-1.3,3.5));
#4707=CARTESIAN_POINT('',(15.6,-1.3,3.5));
#4708=CARTESIAN_POINT('Origin',(15.3,-1.3,2.));
#4709=CARTESIAN_POINT('',(15.,-1.3,0.6));
#4710=CARTESIAN_POINT('',(15.,-1.3,3.5));
#4711=CARTESIAN_POINT('',(15.6,-1.3,0.6));
#4712=CARTESIAN_POINT('',(15.525,-1.3,0.6));
#4713=CARTESIAN_POINT('',(15.6,-1.3,0.5));
#4714=CARTESIAN_POINT('Origin',(15.6,-1.3,3.5));
#4715=CARTESIAN_POINT('',(15.6,-0.65,0.6));
#4716=CARTESIAN_POINT('Origin',(15.,-1.3,0.5));
#4717=CARTESIAN_POINT('',(15.,-0.65,0.6));
#4718=CARTESIAN_POINT('Origin',(17.5,1.8,0.));
#4719=CARTESIAN_POINT('',(17.5,1.8,0.));
#4720=CARTESIAN_POINT('',(14.,1.8,0.));
#4721=CARTESIAN_POINT('',(17.5,1.8,0.));
#4722=CARTESIAN_POINT('',(14.,1.8,0.6));
#4723=CARTESIAN_POINT('',(14.,1.8,0.));
#4724=CARTESIAN_POINT('',(17.5,1.8,0.6));
#4725=CARTESIAN_POINT('',(17.5,1.8,0.6));
#4726=CARTESIAN_POINT('',(17.5,1.8,0.));
#4727=CARTESIAN_POINT('Origin',(17.5,-1.8,0.));
#4728=CARTESIAN_POINT('',(17.5,-1.8,0.));
#4729=CARTESIAN_POINT('',(17.5,-1.8,0.));
#4730=CARTESIAN_POINT('',(17.5,-1.8,0.6));
#4731=CARTESIAN_POINT('',(17.5,-1.8,0.6));
#4732=CARTESIAN_POINT('',(17.5,-1.8,0.));
#4733=CARTESIAN_POINT('Origin',(14.,-1.8,0.));
#4734=CARTESIAN_POINT('',(14.,-1.8,0.));
#4735=CARTESIAN_POINT('',(14.,-1.8,0.));
#4736=CARTESIAN_POINT('',(14.,-1.8,0.6));
#4737=CARTESIAN_POINT('',(14.,-1.8,0.6));
#4738=CARTESIAN_POINT('',(14.,-1.8,0.));
#4739=CARTESIAN_POINT('Origin',(14.,1.8,0.));
#4740=CARTESIAN_POINT('',(14.,1.8,0.));
#4741=CARTESIAN_POINT('',(14.,1.8,0.6));
#4742=CARTESIAN_POINT('Origin',(15.75,0.,0.6));
#4743=CARTESIAN_POINT('Origin',(15.75,0.,0.));
#5417=UNCERTAINTY_MEASURE_WITH_UNIT(LENGTH_MEASURE(0.001),#5459,
'DISTANCE_ACCURACY_VALUE',
'Maximum model space distance between geometric entities at asserted c
onnectivities');
#5435=UNCERTAINTY_MEASURE_WITH_UNIT(LENGTH_MEASURE(0.001),#5459,
'DISTANCE_ACCURACY_VALUE',
'Maximum model space distance between geometric entities at asserted c
onnectivities');
#5440=(
GEOMETRIC_REPRESENTATION_CONTEXT(3)
GLOBAL_UNCERTAINTY_ASSIGNED_CONTEXT((#5417))
GLOBAL_UNIT_ASSIGNED_CONTEXT((#5459,#5461,#5462))
REPRESENTATION_CONTEXT('','3D')
);
#5458=(
GEOMETRIC_REPRESENTATION_CONTEXT(3)
GLOBAL_UNCERTAINTY_ASSIGNED_CONTEXT((#5435))
GLOBAL_UNIT_ASSIGNED_CONTEXT((#5459,#5461,#5462))
REPRESENTATION_CONTEXT('','3D')
);
#5459=(
LENGTH_UNIT()
NAMED_UNIT(*)
SI_UNIT(.CENTI.,.METRE.)
);
#5461=(
NAMED_UNIT(*)
PLANE_ANGLE_UNIT()
SI_UNIT($,.RADIAN.)
);
#5462=(
NAMED_UNIT(*)
SI_UNIT($,.STERADIAN.)
SOLID_ANGLE_UNIT()
);
#5467=SHAPE_DEFINITION_REPRESENTATION(#5489,#5538);
#5489=PRODUCT_DEFINITION_SHAPE('',$,#5561);
#5538=SHAPE_REPRESENTATION('',(#3237),#5440);
#5556=PRODUCT_DEFINITION_CONTEXT('part definition',#5624,'design');
#5561=PRODUCT_DEFINITION('Forked hook catch','Forked hook catch',#5583,
#5556);
#5583=PRODUCT_DEFINITION_FORMATION('',$,#5630);
#5624=APPLICATION_CONTEXT(
'Core Data for Automotive Mechanical Design Process');
#5625=PRODUCT_CONTEXT('part definition',#5624,'mechanical');
#5630=PRODUCT('Forked hook catch','Forked hook catch',
'Forked hook catch',(#5625));
#5725=COLOUR_RGB('Off White',0.89,0.88,0.83);
#5726=FILL_AREA_STYLE_COLOUR('',#5725);
#5727=FILL_AREA_STYLE('',(#5726));
#5728=SURFACE_STYLE_FILL_AREA(#5727);
#5729=SURFACE_SIDE_STYLE('',(#5728));
#5730=SURFACE_STYLE_USAGE(.BOTH.,#5729);
#5731=PRESENTATION_STYLE_ASSIGNMENT((#5730));
ENDSEC;
END-ISO-10303-21;
